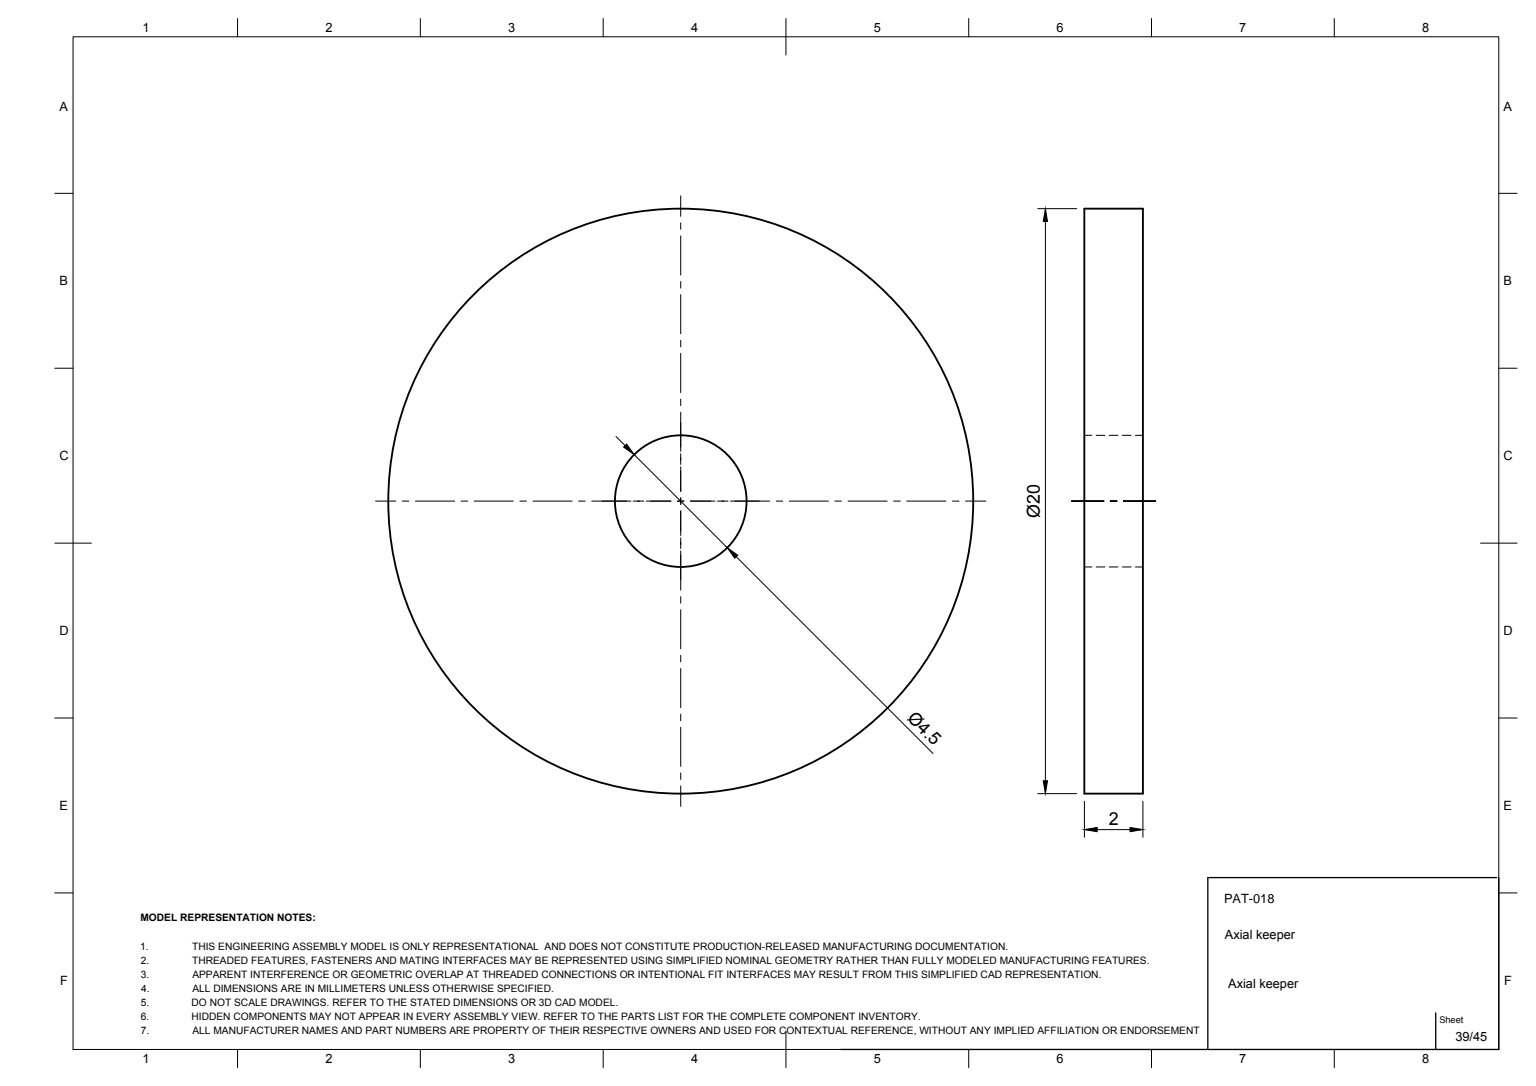
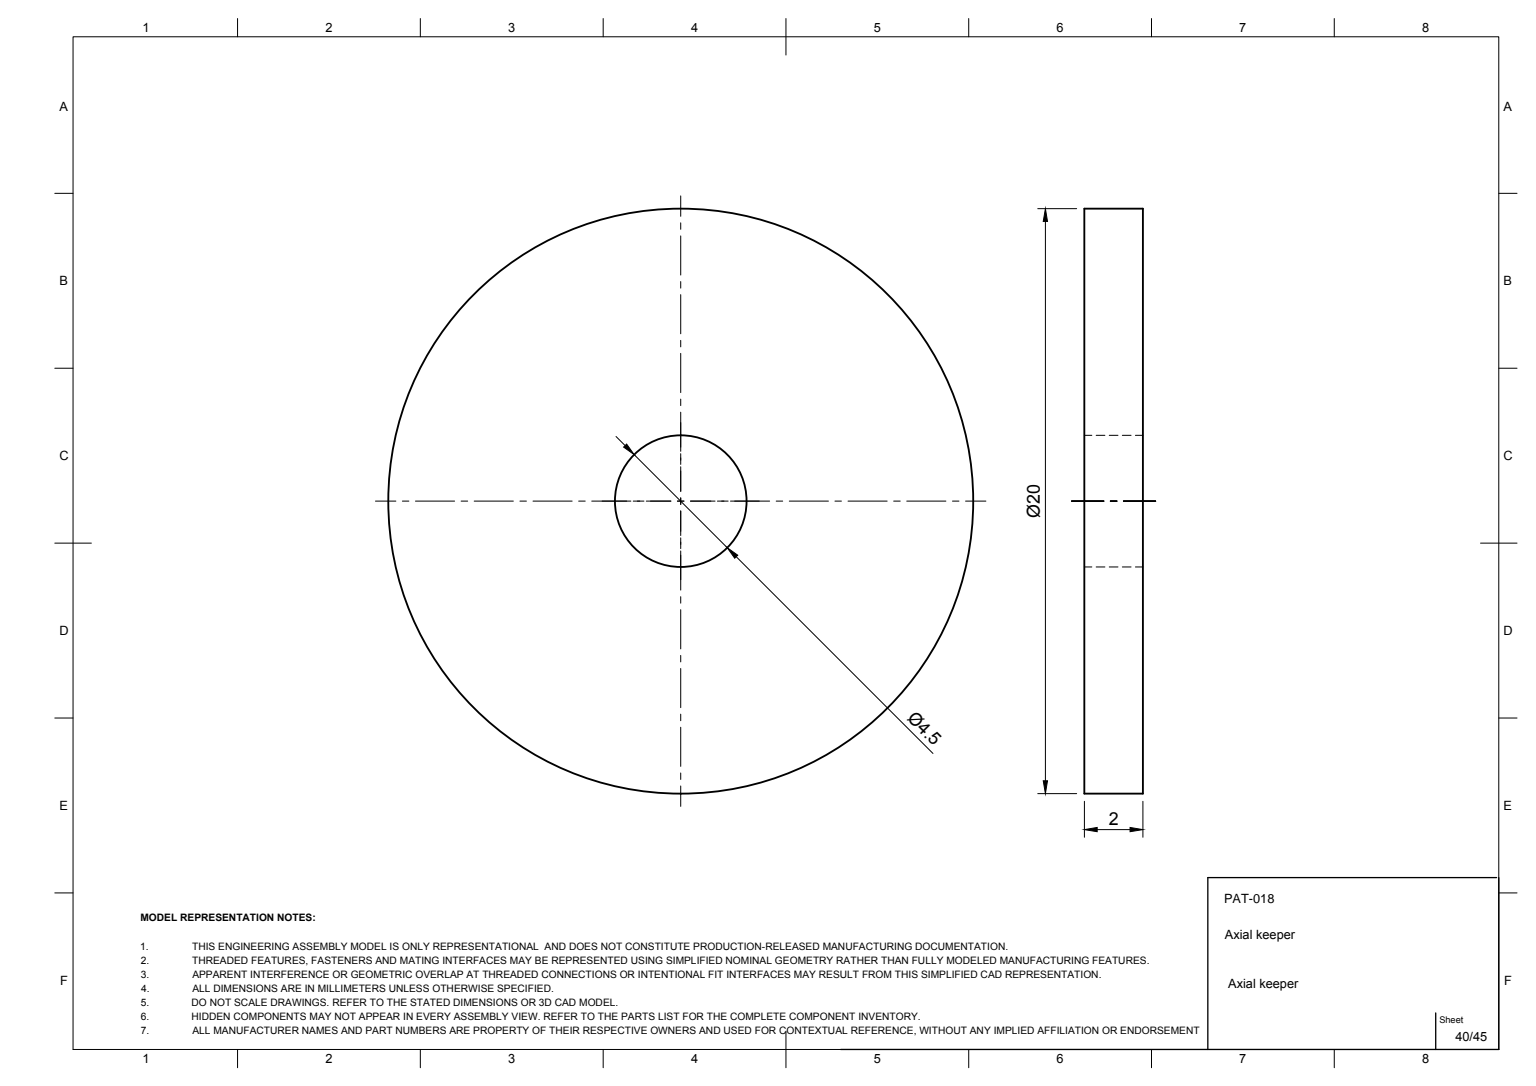
ISO-10303-21;
HEADER;
/* Generated by software containing ST-Developer
 * from STEP Tools, Inc. (www.steptools.com) 
 */

FILE_DESCRIPTION(
/* description */ ('Cam-driven reciprocating slide'),
/* implementation_level */ '2;1');

FILE_NAME(
/* name */ 'Axial keeper.step',
/* time_stamp */ '2026-10-28T03:25:20-07:00',
/* author */ (''),
/* organization */ (''),
/* preprocessor_version */ 'ST-DEVELOPER v20.2',
/* originating_system */ 'Autodesk Translation Framework v15.17.0.0',
/* authorisation */ '');

FILE_SCHEMA (('AUTOMOTIVE_DESIGN { 1 0 10303 214 3 1 1 }'));
ENDSEC;

DATA;
#10=MECHANICAL_DESIGN_GEOMETRIC_PRESENTATION_REPRESENTATION('',(#459),#13277);
#378=SHAPE_REPRESENTATION_RELATIONSHIP('SRR','None',#13474,#415);
#415=ADVANCED_BREP_SHAPE_REPRESENTATION('',(#501),#13269);
#459=STYLED_ITEM('',(#13706),#501);
#501=MANIFOLD_SOLID_BREP('Body1',#6437);
#662=FACE_BOUND('',#1757,.T.);
#663=FACE_BOUND('',#1759,.T.);
#860=PLANE('',#7510);
#861=PLANE('',#7511);
#1220=FACE_OUTER_BOUND('',#1754,.T.);
#1221=FACE_OUTER_BOUND('',#1755,.T.);
#1222=FACE_OUTER_BOUND('',#1756,.T.);
#1223=FACE_OUTER_BOUND('',#1758,.T.);
#1754=EDGE_LOOP('',(#5654,#5655,#5656,#5657));
#1755=EDGE_LOOP('',(#5658,#5659,#5660,#5661));
#1756=EDGE_LOOP('',(#5662));
#1757=EDGE_LOOP('',(#5663));
#1758=EDGE_LOOP('',(#5664));
#1759=EDGE_LOOP('',(#5665));
#2187=LINE('',#12866,#2626);
#2188=LINE('',#12872,#2627);
#2626=VECTOR('',#9329,0.225);
#2627=VECTOR('',#9336,1.);
#3001=CIRCLE('',#7505,0.225);
#3002=CIRCLE('',#7506,0.225);
#3003=CIRCLE('',#7508,1.);
#3004=CIRCLE('',#7509,1.);
#3480=VERTEX_POINT('',#12863);
#3481=VERTEX_POINT('',#12865);
#3482=VERTEX_POINT('',#12869);
#3483=VERTEX_POINT('',#12871);
#4217=EDGE_CURVE('',#3480,#3480,#3001,.T.);
#4218=EDGE_CURVE('',#3480,#3481,#2187,.T.);
#4219=EDGE_CURVE('',#3481,#3481,#3002,.T.);
#4220=EDGE_CURVE('',#3482,#3482,#3003,.T.);
#4221=EDGE_CURVE('',#3482,#3483,#2188,.T.);
#4222=EDGE_CURVE('',#3483,#3483,#3004,.T.);
#5654=ORIENTED_EDGE('',*,*,#4217,.F.);
#5655=ORIENTED_EDGE('',*,*,#4218,.T.);
#5656=ORIENTED_EDGE('',*,*,#4219,.T.);
#5657=ORIENTED_EDGE('',*,*,#4218,.F.);
#5658=ORIENTED_EDGE('',*,*,#4220,.F.);
#5659=ORIENTED_EDGE('',*,*,#4221,.T.);
#5660=ORIENTED_EDGE('',*,*,#4222,.T.);
#5661=ORIENTED_EDGE('',*,*,#4221,.F.);
#5662=ORIENTED_EDGE('',*,*,#4220,.T.);
#5663=ORIENTED_EDGE('',*,*,#4217,.T.);
#5664=ORIENTED_EDGE('',*,*,#4222,.F.);
#5665=ORIENTED_EDGE('',*,*,#4219,.F.);
#6004=CYLINDRICAL_SURFACE('',#7504,0.225);
#6005=CYLINDRICAL_SURFACE('',#7507,1.);
#6338=ADVANCED_FACE('',(#1220),#6004,.F.);
#6339=ADVANCED_FACE('',(#1221),#6005,.T.);
#6340=ADVANCED_FACE('',(#1222,#662),#860,.T.);
#6341=ADVANCED_FACE('',(#1223,#663),#861,.F.);
#6437=CLOSED_SHELL('',(#6338,#6339,#6340,#6341));
#7503=AXIS2_PLACEMENT_3D('',#12861,#9323,#9324);
#7504=AXIS2_PLACEMENT_3D('',#12862,#9325,#9326);
#7505=AXIS2_PLACEMENT_3D('',#12864,#9327,#9328);
#7506=AXIS2_PLACEMENT_3D('',#12867,#9330,#9331);
#7507=AXIS2_PLACEMENT_3D('',#12868,#9332,#9333);
#7508=AXIS2_PLACEMENT_3D('',#12870,#9334,#9335);
#7509=AXIS2_PLACEMENT_3D('',#12873,#9337,#9338);
#7510=AXIS2_PLACEMENT_3D('',#12874,#9339,#9340);
#7511=AXIS2_PLACEMENT_3D('',#12875,#9341,#9342);
#9323=DIRECTION('axis',(0.,0.,1.));
#9324=DIRECTION('refdir',(1.,0.,0.));
#9325=DIRECTION('center_axis',(0.,1.,0.));
#9326=DIRECTION('ref_axis',(1.,0.,0.));
#9327=DIRECTION('center_axis',(0.,-1.,0.));
#9328=DIRECTION('ref_axis',(1.,0.,0.));
#9329=DIRECTION('',(0.,-1.,0.));
#9330=DIRECTION('center_axis',(0.,-1.,0.));
#9331=DIRECTION('ref_axis',(1.,0.,0.));
#9332=DIRECTION('center_axis',(0.,1.,0.));
#9333=DIRECTION('ref_axis',(1.,0.,0.));
#9334=DIRECTION('center_axis',(0.,1.,0.));
#9335=DIRECTION('ref_axis',(1.,0.,0.));
#9336=DIRECTION('',(0.,-1.,0.));
#9337=DIRECTION('center_axis',(0.,1.,0.));
#9338=DIRECTION('ref_axis',(1.,0.,0.));
#9339=DIRECTION('center_axis',(0.,1.,0.));
#9340=DIRECTION('ref_axis',(1.,0.,0.));
#9341=DIRECTION('center_axis',(0.,1.,0.));
#9342=DIRECTION('ref_axis',(1.,0.,0.));
#12861=CARTESIAN_POINT('',(0.,0.,0.));
#12862=CARTESIAN_POINT('Origin',(0.,-4.7,4.));
#12863=CARTESIAN_POINT('',(-0.225,-4.5,4.));
#12864=CARTESIAN_POINT('Origin',(0.,-4.5,4.));
#12865=CARTESIAN_POINT('',(-0.225,-4.7,4.));
#12866=CARTESIAN_POINT('',(-0.225,-4.7,4.));
#12867=CARTESIAN_POINT('Origin',(0.,-4.7,4.));
#12868=CARTESIAN_POINT('Origin',(0.,-4.7,4.));
#12869=CARTESIAN_POINT('',(-1.,-4.5,4.));
#12870=CARTESIAN_POINT('Origin',(0.,-4.5,4.));
#12871=CARTESIAN_POINT('',(-1.,-4.7,4.));
#12872=CARTESIAN_POINT('',(-1.,-4.7,4.));
#12873=CARTESIAN_POINT('Origin',(0.,-4.7,4.));
#12874=CARTESIAN_POINT('Origin',(0.,-4.5,4.));
#12875=CARTESIAN_POINT('Origin',(0.,-4.7,4.));
#13225=UNCERTAINTY_MEASURE_WITH_UNIT(LENGTH_MEASURE(0.001),#13278,
'DISTANCE_ACCURACY_VALUE',
'Maximum model space distance between geometric entities at asserted c
onnectivities');
#13233=UNCERTAINTY_MEASURE_WITH_UNIT(LENGTH_MEASURE(0.001),#13278,
'DISTANCE_ACCURACY_VALUE',
'Maximum model space distance between geometric entities at asserted c
onnectivities');
#13269=(
GEOMETRIC_REPRESENTATION_CONTEXT(3)
GLOBAL_UNCERTAINTY_ASSIGNED_CONTEXT((#13225))
GLOBAL_UNIT_ASSIGNED_CONTEXT((#13278,#13280,#13281))
REPRESENTATION_CONTEXT('','3D')
);
#13277=(
GEOMETRIC_REPRESENTATION_CONTEXT(3)
GLOBAL_UNCERTAINTY_ASSIGNED_CONTEXT((#13233))
GLOBAL_UNIT_ASSIGNED_CONTEXT((#13278,#13280,#13281))
REPRESENTATION_CONTEXT('','3D')
);
#13278=(
LENGTH_UNIT()
NAMED_UNIT(*)
SI_UNIT(.CENTI.,.METRE.)
);
#13280=(
NAMED_UNIT(*)
PLANE_ANGLE_UNIT()
SI_UNIT($,.RADIAN.)
);
#13281=(
NAMED_UNIT(*)
SI_UNIT($,.STERADIAN.)
SOLID_ANGLE_UNIT()
);
#13317=SHAPE_DEFINITION_REPRESENTATION(#13367,#13474);
#13367=PRODUCT_DEFINITION_SHAPE('',$,#13518);
#13474=SHAPE_REPRESENTATION('',(#7503),#13269);
#13482=PRODUCT_DEFINITION_CONTEXT('part definition',#13613,'design');
#13518=PRODUCT_DEFINITION('Axial keeper','Axial keeper',#13561,#13482);
#13561=PRODUCT_DEFINITION_FORMATION('',$,#13650);
#13613=APPLICATION_CONTEXT(
'Core Data for Automotive Mechanical Design Process');
#13614=PRODUCT_CONTEXT('part definition',#13613,'mechanical');
#13650=PRODUCT('Axial keeper','Axial keeper','Axial keeper',(#13614));
#13700=COLOUR_RGB('Light Blue',0.38,0.62,0.78);
#13701=FILL_AREA_STYLE_COLOUR('',#13700);
#13702=FILL_AREA_STYLE('',(#13701));
#13703=SURFACE_STYLE_FILL_AREA(#13702);
#13704=SURFACE_SIDE_STYLE('',(#13703));
#13705=SURFACE_STYLE_USAGE(.BOTH.,#13704);
#13706=PRESENTATION_STYLE_ASSIGNMENT((#13705));
ENDSEC;
END-ISO-10303-21;
